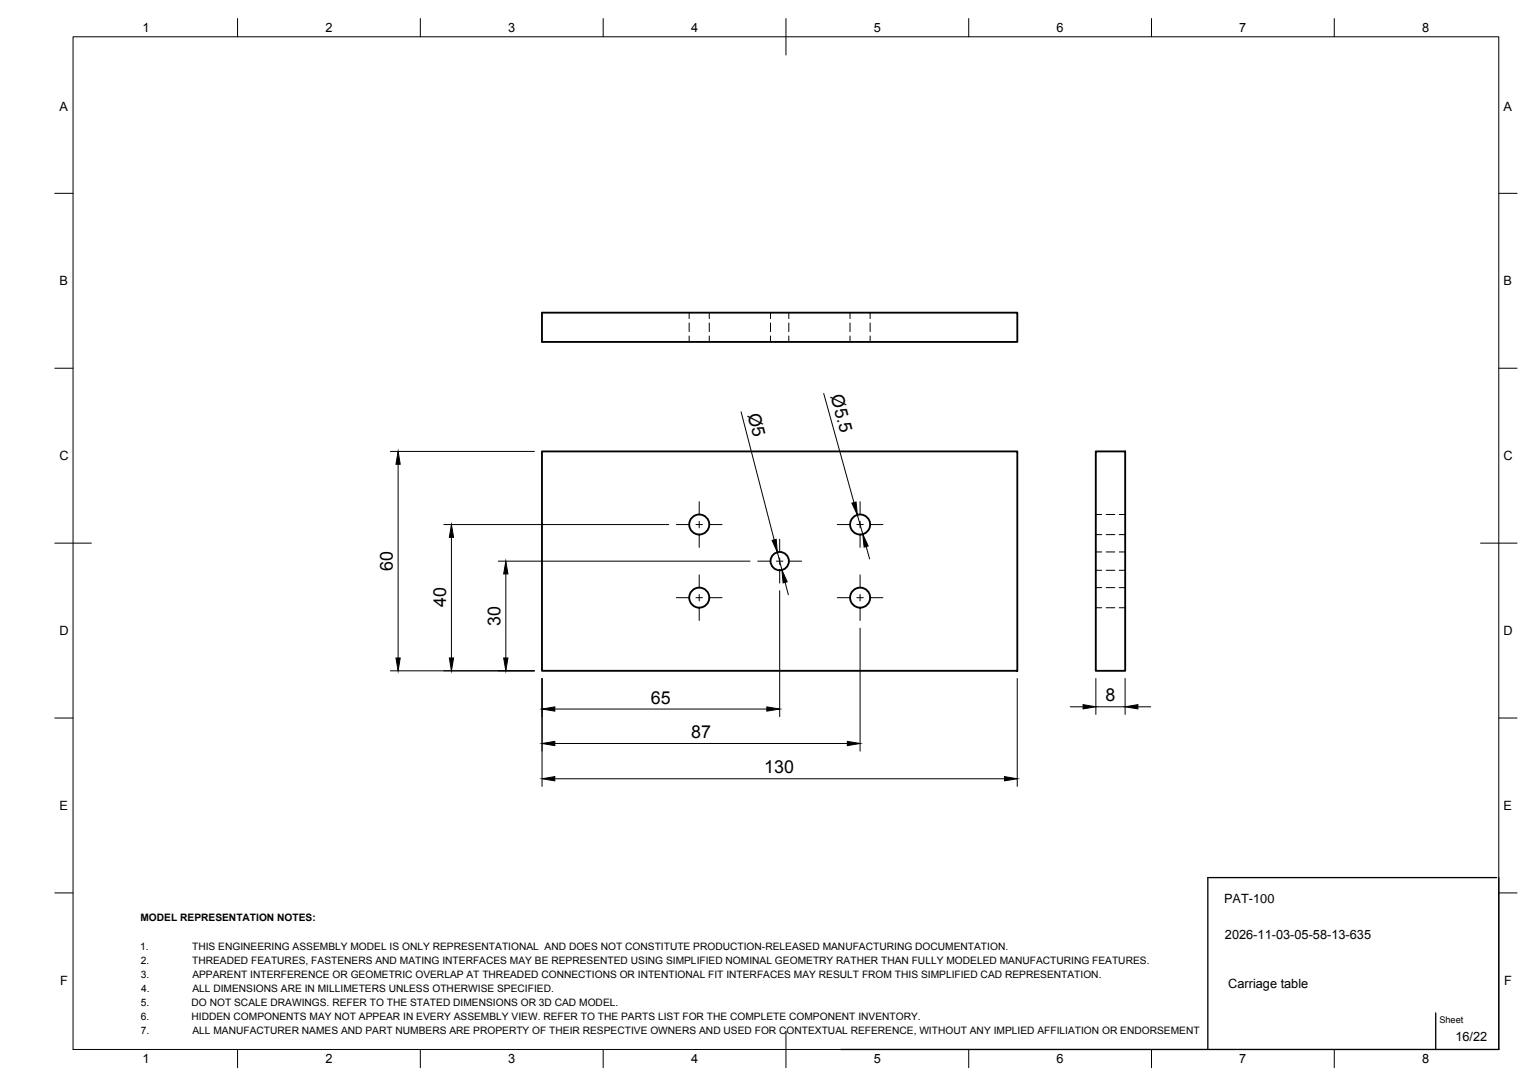
ISO-10303-21;
HEADER;
/* Generated by software containing ST-Developer
 * from STEP Tools, Inc. (www.steptools.com) 
 */

FILE_DESCRIPTION(
/* description */ (''),
/* implementation_level */ '2;1');

FILE_NAME(
/* name */ 'Carriage table.step',
/* time_stamp */ '2026-10-29T16:43:51-07:00',
/* author */ (''),
/* organization */ (''),
/* preprocessor_version */ 'ST-DEVELOPER v20.2',
/* originating_system */ 'Autodesk Translation Framework v15.17.0.0',
/* authorisation */ '');

FILE_SCHEMA (('AUTOMOTIVE_DESIGN { 1 0 10303 214 3 1 1 }'));
ENDSEC;

DATA;
#10=MECHANICAL_DESIGN_GEOMETRIC_PRESENTATION_REPRESENTATION('',(#379),#10292);
#333=SHAPE_REPRESENTATION_RELATIONSHIP('SRR','None',#10430,#356);
#356=ADVANCED_BREP_SHAPE_REPRESENTATION('',(#400),#10282);
#379=STYLED_ITEM('',(#10621),#400);
#400=MANIFOLD_SOLID_BREP('Body1',#5023);
#491=FACE_BOUND('',#1274,.T.);
#492=FACE_BOUND('',#1275,.T.);
#493=FACE_BOUND('',#1276,.T.);
#494=FACE_BOUND('',#1277,.T.);
#495=FACE_BOUND('',#1278,.T.);
#496=FACE_BOUND('',#1280,.T.);
#497=FACE_BOUND('',#1281,.T.);
#498=FACE_BOUND('',#1282,.T.);
#499=FACE_BOUND('',#1283,.T.);
#500=FACE_BOUND('',#1284,.T.);
#644=PLANE('',#5625);
#645=PLANE('',#5626);
#646=PLANE('',#5627);
#647=PLANE('',#5628);
#648=PLANE('',#5629);
#649=PLANE('',#5630);
#891=FACE_OUTER_BOUND('',#1264,.T.);
#892=FACE_OUTER_BOUND('',#1265,.T.);
#893=FACE_OUTER_BOUND('',#1266,.T.);
#894=FACE_OUTER_BOUND('',#1267,.T.);
#895=FACE_OUTER_BOUND('',#1268,.T.);
#896=FACE_OUTER_BOUND('',#1269,.T.);
#897=FACE_OUTER_BOUND('',#1270,.T.);
#898=FACE_OUTER_BOUND('',#1271,.T.);
#899=FACE_OUTER_BOUND('',#1272,.T.);
#900=FACE_OUTER_BOUND('',#1273,.T.);
#901=FACE_OUTER_BOUND('',#1279,.T.);
#1264=EDGE_LOOP('',(#4211,#4212,#4213,#4214));
#1265=EDGE_LOOP('',(#4215,#4216,#4217,#4218));
#1266=EDGE_LOOP('',(#4219,#4220,#4221,#4222));
#1267=EDGE_LOOP('',(#4223,#4224,#4225,#4226));
#1268=EDGE_LOOP('',(#4227,#4228,#4229,#4230));
#1269=EDGE_LOOP('',(#4231,#4232,#4233,#4234));
#1270=EDGE_LOOP('',(#4235,#4236,#4237,#4238));
#1271=EDGE_LOOP('',(#4239,#4240,#4241,#4242));
#1272=EDGE_LOOP('',(#4243,#4244,#4245,#4246));
#1273=EDGE_LOOP('',(#4247,#4248,#4249,#4250));
#1274=EDGE_LOOP('',(#4251));
#1275=EDGE_LOOP('',(#4252));
#1276=EDGE_LOOP('',(#4253));
#1277=EDGE_LOOP('',(#4254));
#1278=EDGE_LOOP('',(#4255));
#1279=EDGE_LOOP('',(#4256,#4257,#4258,#4259));
#1280=EDGE_LOOP('',(#4260));
#1281=EDGE_LOOP('',(#4261));
#1282=EDGE_LOOP('',(#4262));
#1283=EDGE_LOOP('',(#4263));
#1284=EDGE_LOOP('',(#4264));
#1666=LINE('',#9712,#2058);
#1667=LINE('',#9718,#2059);
#1668=LINE('',#9724,#2060);
#1669=LINE('',#9730,#2061);
#1670=LINE('',#9736,#2062);
#1671=LINE('',#9741,#2063);
#1672=LINE('',#9743,#2064);
#1673=LINE('',#9745,#2065);
#1674=LINE('',#9746,#2066);
#1675=LINE('',#9749,#2067);
#1676=LINE('',#9751,#2068);
#1677=LINE('',#9752,#2069);
#1678=LINE('',#9755,#2070);
#1679=LINE('',#9757,#2071);
#1680=LINE('',#9758,#2072);
#1681=LINE('',#9760,#2073);
#1682=LINE('',#9761,#2074);
#2058=VECTOR('',#6765,0.25);
#2059=VECTOR('',#6772,0.274999999999999);
#2060=VECTOR('',#6779,0.275);
#2061=VECTOR('',#6786,0.275);
#2062=VECTOR('',#6793,0.274999999999999);
#2063=VECTOR('',#6798,1.);
#2064=VECTOR('',#6799,1.);
#2065=VECTOR('',#6800,1.);
#2066=VECTOR('',#6801,1.);
#2067=VECTOR('',#6804,1.);
#2068=VECTOR('',#6805,1.);
#2069=VECTOR('',#6806,1.);
#2070=VECTOR('',#6809,1.);
#2071=VECTOR('',#6810,1.);
#2072=VECTOR('',#6811,1.);
#2073=VECTOR('',#6814,1.);
#2074=VECTOR('',#6815,1.);
#2318=CIRCLE('',#5611,0.25);
#2319=CIRCLE('',#5612,0.25);
#2320=CIRCLE('',#5614,0.274999999999999);
#2321=CIRCLE('',#5615,0.274999999999999);
#2322=CIRCLE('',#5617,0.275);
#2323=CIRCLE('',#5618,0.275);
#2324=CIRCLE('',#5620,0.275);
#2325=CIRCLE('',#5621,0.275);
#2326=CIRCLE('',#5623,0.274999999999999);
#2327=CIRCLE('',#5624,0.274999999999999);
#2657=VERTEX_POINT('',#9709);
#2658=VERTEX_POINT('',#9711);
#2659=VERTEX_POINT('',#9715);
#2660=VERTEX_POINT('',#9717);
#2661=VERTEX_POINT('',#9721);
#2662=VERTEX_POINT('',#9723);
#2663=VERTEX_POINT('',#9727);
#2664=VERTEX_POINT('',#9729);
#2665=VERTEX_POINT('',#9733);
#2666=VERTEX_POINT('',#9735);
#2667=VERTEX_POINT('',#9739);
#2668=VERTEX_POINT('',#9740);
#2669=VERTEX_POINT('',#9742);
#2670=VERTEX_POINT('',#9744);
#2671=VERTEX_POINT('',#9748);
#2672=VERTEX_POINT('',#9750);
#2673=VERTEX_POINT('',#9754);
#2674=VERTEX_POINT('',#9756);
#3196=EDGE_CURVE('',#2657,#2657,#2318,.T.);
#3197=EDGE_CURVE('',#2657,#2658,#1666,.T.);
#3198=EDGE_CURVE('',#2658,#2658,#2319,.T.);
#3199=EDGE_CURVE('',#2659,#2659,#2320,.T.);
#3200=EDGE_CURVE('',#2659,#2660,#1667,.T.);
#3201=EDGE_CURVE('',#2660,#2660,#2321,.T.);
#3202=EDGE_CURVE('',#2661,#2661,#2322,.T.);
#3203=EDGE_CURVE('',#2661,#2662,#1668,.T.);
#3204=EDGE_CURVE('',#2662,#2662,#2323,.T.);
#3205=EDGE_CURVE('',#2663,#2663,#2324,.T.);
#3206=EDGE_CURVE('',#2663,#2664,#1669,.T.);
#3207=EDGE_CURVE('',#2664,#2664,#2325,.T.);
#3208=EDGE_CURVE('',#2665,#2665,#2326,.T.);
#3209=EDGE_CURVE('',#2665,#2666,#1670,.T.);
#3210=EDGE_CURVE('',#2666,#2666,#2327,.T.);
#3211=EDGE_CURVE('',#2667,#2668,#1671,.T.);
#3212=EDGE_CURVE('',#2668,#2669,#1672,.T.);
#3213=EDGE_CURVE('',#2670,#2669,#1673,.T.);
#3214=EDGE_CURVE('',#2667,#2670,#1674,.T.);
#3215=EDGE_CURVE('',#2671,#2667,#1675,.T.);
#3216=EDGE_CURVE('',#2672,#2670,#1676,.T.);
#3217=EDGE_CURVE('',#2671,#2672,#1677,.T.);
#3218=EDGE_CURVE('',#2673,#2671,#1678,.T.);
#3219=EDGE_CURVE('',#2674,#2672,#1679,.T.);
#3220=EDGE_CURVE('',#2673,#2674,#1680,.T.);
#3221=EDGE_CURVE('',#2668,#2673,#1681,.T.);
#3222=EDGE_CURVE('',#2669,#2674,#1682,.T.);
#4211=ORIENTED_EDGE('',*,*,#3196,.F.);
#4212=ORIENTED_EDGE('',*,*,#3197,.T.);
#4213=ORIENTED_EDGE('',*,*,#3198,.F.);
#4214=ORIENTED_EDGE('',*,*,#3197,.F.);
#4215=ORIENTED_EDGE('',*,*,#3199,.F.);
#4216=ORIENTED_EDGE('',*,*,#3200,.T.);
#4217=ORIENTED_EDGE('',*,*,#3201,.F.);
#4218=ORIENTED_EDGE('',*,*,#3200,.F.);
#4219=ORIENTED_EDGE('',*,*,#3202,.F.);
#4220=ORIENTED_EDGE('',*,*,#3203,.T.);
#4221=ORIENTED_EDGE('',*,*,#3204,.F.);
#4222=ORIENTED_EDGE('',*,*,#3203,.F.);
#4223=ORIENTED_EDGE('',*,*,#3205,.F.);
#4224=ORIENTED_EDGE('',*,*,#3206,.T.);
#4225=ORIENTED_EDGE('',*,*,#3207,.F.);
#4226=ORIENTED_EDGE('',*,*,#3206,.F.);
#4227=ORIENTED_EDGE('',*,*,#3208,.F.);
#4228=ORIENTED_EDGE('',*,*,#3209,.T.);
#4229=ORIENTED_EDGE('',*,*,#3210,.F.);
#4230=ORIENTED_EDGE('',*,*,#3209,.F.);
#4231=ORIENTED_EDGE('',*,*,#3211,.T.);
#4232=ORIENTED_EDGE('',*,*,#3212,.T.);
#4233=ORIENTED_EDGE('',*,*,#3213,.F.);
#4234=ORIENTED_EDGE('',*,*,#3214,.F.);
#4235=ORIENTED_EDGE('',*,*,#3215,.T.);
#4236=ORIENTED_EDGE('',*,*,#3214,.T.);
#4237=ORIENTED_EDGE('',*,*,#3216,.F.);
#4238=ORIENTED_EDGE('',*,*,#3217,.F.);
#4239=ORIENTED_EDGE('',*,*,#3218,.T.);
#4240=ORIENTED_EDGE('',*,*,#3217,.T.);
#4241=ORIENTED_EDGE('',*,*,#3219,.F.);
#4242=ORIENTED_EDGE('',*,*,#3220,.F.);
#4243=ORIENTED_EDGE('',*,*,#3221,.T.);
#4244=ORIENTED_EDGE('',*,*,#3220,.T.);
#4245=ORIENTED_EDGE('',*,*,#3222,.F.);
#4246=ORIENTED_EDGE('',*,*,#3212,.F.);
#4247=ORIENTED_EDGE('',*,*,#3222,.T.);
#4248=ORIENTED_EDGE('',*,*,#3219,.T.);
#4249=ORIENTED_EDGE('',*,*,#3216,.T.);
#4250=ORIENTED_EDGE('',*,*,#3213,.T.);
#4251=ORIENTED_EDGE('',*,*,#3198,.T.);
#4252=ORIENTED_EDGE('',*,*,#3201,.T.);
#4253=ORIENTED_EDGE('',*,*,#3204,.T.);
#4254=ORIENTED_EDGE('',*,*,#3207,.T.);
#4255=ORIENTED_EDGE('',*,*,#3210,.T.);
#4256=ORIENTED_EDGE('',*,*,#3221,.F.);
#4257=ORIENTED_EDGE('',*,*,#3211,.F.);
#4258=ORIENTED_EDGE('',*,*,#3215,.F.);
#4259=ORIENTED_EDGE('',*,*,#3218,.F.);
#4260=ORIENTED_EDGE('',*,*,#3196,.T.);
#4261=ORIENTED_EDGE('',*,*,#3199,.T.);
#4262=ORIENTED_EDGE('',*,*,#3202,.T.);
#4263=ORIENTED_EDGE('',*,*,#3205,.T.);
#4264=ORIENTED_EDGE('',*,*,#3208,.T.);
#4690=CYLINDRICAL_SURFACE('',#5610,0.25);
#4691=CYLINDRICAL_SURFACE('',#5613,0.274999999999999);
#4692=CYLINDRICAL_SURFACE('',#5616,0.275);
#4693=CYLINDRICAL_SURFACE('',#5619,0.275);
#4694=CYLINDRICAL_SURFACE('',#5622,0.274999999999999);
#4900=ADVANCED_FACE('',(#891),#4690,.F.);
#4901=ADVANCED_FACE('',(#892),#4691,.F.);
#4902=ADVANCED_FACE('',(#893),#4692,.F.);
#4903=ADVANCED_FACE('',(#894),#4693,.F.);
#4904=ADVANCED_FACE('',(#895),#4694,.F.);
#4905=ADVANCED_FACE('',(#896),#644,.T.);
#4906=ADVANCED_FACE('',(#897),#645,.T.);
#4907=ADVANCED_FACE('',(#898),#646,.T.);
#4908=ADVANCED_FACE('',(#899),#647,.T.);
#4909=ADVANCED_FACE('',(#900,#491,#492,#493,#494,#495),#648,.T.);
#4910=ADVANCED_FACE('',(#901,#496,#497,#498,#499,#500),#649,.F.);
#5023=CLOSED_SHELL('',(#4900,#4901,#4902,#4903,#4904,#4905,#4906,#4907,
#4908,#4909,#4910));
#5609=AXIS2_PLACEMENT_3D('',#9707,#6759,#6760);
#5610=AXIS2_PLACEMENT_3D('',#9708,#6761,#6762);
#5611=AXIS2_PLACEMENT_3D('',#9710,#6763,#6764);
#5612=AXIS2_PLACEMENT_3D('',#9713,#6766,#6767);
#5613=AXIS2_PLACEMENT_3D('',#9714,#6768,#6769);
#5614=AXIS2_PLACEMENT_3D('',#9716,#6770,#6771);
#5615=AXIS2_PLACEMENT_3D('',#9719,#6773,#6774);
#5616=AXIS2_PLACEMENT_3D('',#9720,#6775,#6776);
#5617=AXIS2_PLACEMENT_3D('',#9722,#6777,#6778);
#5618=AXIS2_PLACEMENT_3D('',#9725,#6780,#6781);
#5619=AXIS2_PLACEMENT_3D('',#9726,#6782,#6783);
#5620=AXIS2_PLACEMENT_3D('',#9728,#6784,#6785);
#5621=AXIS2_PLACEMENT_3D('',#9731,#6787,#6788);
#5622=AXIS2_PLACEMENT_3D('',#9732,#6789,#6790);
#5623=AXIS2_PLACEMENT_3D('',#9734,#6791,#6792);
#5624=AXIS2_PLACEMENT_3D('',#9737,#6794,#6795);
#5625=AXIS2_PLACEMENT_3D('',#9738,#6796,#6797);
#5626=AXIS2_PLACEMENT_3D('',#9747,#6802,#6803);
#5627=AXIS2_PLACEMENT_3D('',#9753,#6807,#6808);
#5628=AXIS2_PLACEMENT_3D('',#9759,#6812,#6813);
#5629=AXIS2_PLACEMENT_3D('',#9762,#6816,#6817);
#5630=AXIS2_PLACEMENT_3D('',#9763,#6818,#6819);
#6759=DIRECTION('axis',(0.,0.,1.));
#6760=DIRECTION('refdir',(1.,0.,0.));
#6761=DIRECTION('center_axis',(0.,0.,1.));
#6762=DIRECTION('ref_axis',(1.,0.,0.));
#6763=DIRECTION('center_axis',(0.,0.,1.));
#6764=DIRECTION('ref_axis',(1.,0.,0.));
#6765=DIRECTION('',(0.,0.,1.));
#6766=DIRECTION('center_axis',(0.,0.,-1.));
#6767=DIRECTION('ref_axis',(1.,0.,0.));
#6768=DIRECTION('center_axis',(0.,0.,1.));
#6769=DIRECTION('ref_axis',(1.,0.,0.));
#6770=DIRECTION('center_axis',(0.,0.,1.));
#6771=DIRECTION('ref_axis',(1.,0.,0.));
#6772=DIRECTION('',(0.,0.,1.));
#6773=DIRECTION('center_axis',(0.,0.,-1.));
#6774=DIRECTION('ref_axis',(1.,0.,0.));
#6775=DIRECTION('center_axis',(0.,0.,1.));
#6776=DIRECTION('ref_axis',(1.,0.,0.));
#6777=DIRECTION('center_axis',(0.,0.,1.));
#6778=DIRECTION('ref_axis',(1.,0.,0.));
#6779=DIRECTION('',(0.,0.,1.));
#6780=DIRECTION('center_axis',(0.,0.,-1.));
#6781=DIRECTION('ref_axis',(1.,0.,0.));
#6782=DIRECTION('center_axis',(0.,0.,1.));
#6783=DIRECTION('ref_axis',(1.,0.,0.));
#6784=DIRECTION('center_axis',(0.,0.,1.));
#6785=DIRECTION('ref_axis',(1.,0.,0.));
#6786=DIRECTION('',(0.,0.,1.));
#6787=DIRECTION('center_axis',(0.,0.,-1.));
#6788=DIRECTION('ref_axis',(1.,0.,0.));
#6789=DIRECTION('center_axis',(0.,0.,1.));
#6790=DIRECTION('ref_axis',(1.,0.,0.));
#6791=DIRECTION('center_axis',(0.,0.,1.));
#6792=DIRECTION('ref_axis',(1.,0.,0.));
#6793=DIRECTION('',(0.,0.,1.));
#6794=DIRECTION('center_axis',(0.,0.,-1.));
#6795=DIRECTION('ref_axis',(1.,0.,0.));
#6796=DIRECTION('center_axis',(0.,1.,0.));
#6797=DIRECTION('ref_axis',(-1.,0.,0.));
#6798=DIRECTION('',(-1.,0.,0.));
#6799=DIRECTION('',(0.,0.,1.));
#6800=DIRECTION('',(-1.,0.,0.));
#6801=DIRECTION('',(0.,0.,1.));
#6802=DIRECTION('center_axis',(1.,0.,0.));
#6803=DIRECTION('ref_axis',(0.,1.,0.));
#6804=DIRECTION('',(0.,1.,0.));
#6805=DIRECTION('',(0.,1.,0.));
#6806=DIRECTION('',(0.,0.,1.));
#6807=DIRECTION('center_axis',(0.,-1.,0.));
#6808=DIRECTION('ref_axis',(1.,0.,0.));
#6809=DIRECTION('',(1.,0.,0.));
#6810=DIRECTION('',(1.,0.,0.));
#6811=DIRECTION('',(0.,0.,1.));
#6812=DIRECTION('center_axis',(-1.,0.,0.));
#6813=DIRECTION('ref_axis',(0.,-1.,0.));
#6814=DIRECTION('',(0.,-1.,0.));
#6815=DIRECTION('',(0.,-1.,0.));
#6816=DIRECTION('center_axis',(0.,0.,1.));
#6817=DIRECTION('ref_axis',(1.,0.,0.));
#6818=DIRECTION('center_axis',(0.,0.,1.));
#6819=DIRECTION('ref_axis',(1.,0.,0.));
#9707=CARTESIAN_POINT('',(0.,0.,0.));
#9708=CARTESIAN_POINT('Origin',(15.,0.,5.7));
#9709=CARTESIAN_POINT('',(14.75,-3.06161699786838E-17,5.8));
#9710=CARTESIAN_POINT('Origin',(15.,0.,5.8));
#9711=CARTESIAN_POINT('',(14.75,3.06161699786838E-17,6.6));
#9712=CARTESIAN_POINT('',(14.75,-3.06161699786838E-17,5.7));
#9713=CARTESIAN_POINT('Origin',(15.,0.,6.6));
#9714=CARTESIAN_POINT('Origin',(16.,-2.2,5.7));
#9715=CARTESIAN_POINT('',(15.725,-2.2,5.8));
#9716=CARTESIAN_POINT('Origin',(16.,-2.2,5.8));
#9717=CARTESIAN_POINT('',(15.725,-2.2,6.6));
#9718=CARTESIAN_POINT('',(15.725,-2.2,5.7));
#9719=CARTESIAN_POINT('Origin',(16.,-2.2,6.6));
#9720=CARTESIAN_POINT('Origin',(14.,2.2,5.7));
#9721=CARTESIAN_POINT('',(13.725,2.2,5.8));
#9722=CARTESIAN_POINT('Origin',(14.,2.2,5.8));
#9723=CARTESIAN_POINT('',(13.725,2.2,6.6));
#9724=CARTESIAN_POINT('',(13.725,2.2,5.7));
#9725=CARTESIAN_POINT('Origin',(14.,2.2,6.6));
#9726=CARTESIAN_POINT('Origin',(14.,-2.2,5.7));
#9727=CARTESIAN_POINT('',(13.725,-2.2,5.8));
#9728=CARTESIAN_POINT('Origin',(14.,-2.2,5.8));
#9729=CARTESIAN_POINT('',(13.725,-2.2,6.6));
#9730=CARTESIAN_POINT('',(13.725,-2.2,5.7));
#9731=CARTESIAN_POINT('Origin',(14.,-2.2,6.6));
#9732=CARTESIAN_POINT('Origin',(16.,2.2,5.7));
#9733=CARTESIAN_POINT('',(15.725,2.2,5.8));
#9734=CARTESIAN_POINT('Origin',(16.,2.2,5.8));
#9735=CARTESIAN_POINT('',(15.725,2.2,6.6));
#9736=CARTESIAN_POINT('',(15.725,2.2,5.7));
#9737=CARTESIAN_POINT('Origin',(16.,2.2,6.6));
#9738=CARTESIAN_POINT('Origin',(18.,6.5,5.8));
#9739=CARTESIAN_POINT('',(18.,6.5,5.8));
#9740=CARTESIAN_POINT('',(12.,6.5,5.8));
#9741=CARTESIAN_POINT('',(18.,6.5,5.8));
#9742=CARTESIAN_POINT('',(12.,6.5,6.6));
#9743=CARTESIAN_POINT('',(12.,6.5,5.8));
#9744=CARTESIAN_POINT('',(18.,6.5,6.6));
#9745=CARTESIAN_POINT('',(18.,6.5,6.6));
#9746=CARTESIAN_POINT('',(18.,6.5,5.8));
#9747=CARTESIAN_POINT('Origin',(18.,-6.5,5.8));
#9748=CARTESIAN_POINT('',(18.,-6.5,5.8));
#9749=CARTESIAN_POINT('',(18.,-6.5,5.8));
#9750=CARTESIAN_POINT('',(18.,-6.5,6.6));
#9751=CARTESIAN_POINT('',(18.,-6.5,6.6));
#9752=CARTESIAN_POINT('',(18.,-6.5,5.8));
#9753=CARTESIAN_POINT('Origin',(12.,-6.5,5.8));
#9754=CARTESIAN_POINT('',(12.,-6.5,5.8));
#9755=CARTESIAN_POINT('',(12.,-6.5,5.8));
#9756=CARTESIAN_POINT('',(12.,-6.5,6.6));
#9757=CARTESIAN_POINT('',(12.,-6.5,6.6));
#9758=CARTESIAN_POINT('',(12.,-6.5,5.8));
#9759=CARTESIAN_POINT('Origin',(12.,6.5,5.8));
#9760=CARTESIAN_POINT('',(12.,6.5,5.8));
#9761=CARTESIAN_POINT('',(12.,6.5,6.6));
#9762=CARTESIAN_POINT('Origin',(15.,0.,6.6));
#9763=CARTESIAN_POINT('Origin',(15.,0.,5.8));
#10254=UNCERTAINTY_MEASURE_WITH_UNIT(LENGTH_MEASURE(0.001),#10293,
'DISTANCE_ACCURACY_VALUE',
'Maximum model space distance between geometric entities at asserted c
onnectivities');
#10264=UNCERTAINTY_MEASURE_WITH_UNIT(LENGTH_MEASURE(0.001),#10293,
'DISTANCE_ACCURACY_VALUE',
'Maximum model space distance between geometric entities at asserted c
onnectivities');
#10282=(
GEOMETRIC_REPRESENTATION_CONTEXT(3)
GLOBAL_UNCERTAINTY_ASSIGNED_CONTEXT((#10254))
GLOBAL_UNIT_ASSIGNED_CONTEXT((#10293,#10295,#10296))
REPRESENTATION_CONTEXT('','3D')
);
#10292=(
GEOMETRIC_REPRESENTATION_CONTEXT(3)
GLOBAL_UNCERTAINTY_ASSIGNED_CONTEXT((#10264))
GLOBAL_UNIT_ASSIGNED_CONTEXT((#10293,#10295,#10296))
REPRESENTATION_CONTEXT('','3D')
);
#10293=(
LENGTH_UNIT()
NAMED_UNIT(*)
SI_UNIT(.CENTI.,.METRE.)
);
#10295=(
NAMED_UNIT(*)
PLANE_ANGLE_UNIT()
SI_UNIT($,.RADIAN.)
);
#10296=(
NAMED_UNIT(*)
SI_UNIT($,.STERADIAN.)
SOLID_ANGLE_UNIT()
);
#10314=SHAPE_DEFINITION_REPRESENTATION(#10341,#10430);
#10341=PRODUCT_DEFINITION_SHAPE('',$,#10458);
#10430=SHAPE_REPRESENTATION('',(#5609),#10282);
#10440=PRODUCT_DEFINITION_CONTEXT('part definition',#10523,'design');
#10458=PRODUCT_DEFINITION('Carriage table','Carriage table',#10485,
#10440);
#10485=PRODUCT_DEFINITION_FORMATION('',$,#10542);
#10523=APPLICATION_CONTEXT(
'Core Data for Automotive Mechanical Design Process');
#10524=PRODUCT_CONTEXT('part definition',#10523,'mechanical');
#10542=PRODUCT('Carriage table','Carriage table',
'Carriage table',(#10524));
#10615=COLOUR_RGB('Sky Blue',0.24,0.69,0.87);
#10616=FILL_AREA_STYLE_COLOUR('',#10615);
#10617=FILL_AREA_STYLE('',(#10616));
#10618=SURFACE_STYLE_FILL_AREA(#10617);
#10619=SURFACE_SIDE_STYLE('',(#10618));
#10620=SURFACE_STYLE_USAGE(.BOTH.,#10619);
#10621=PRESENTATION_STYLE_ASSIGNMENT((#10620));
ENDSEC;
END-ISO-10303-21;
